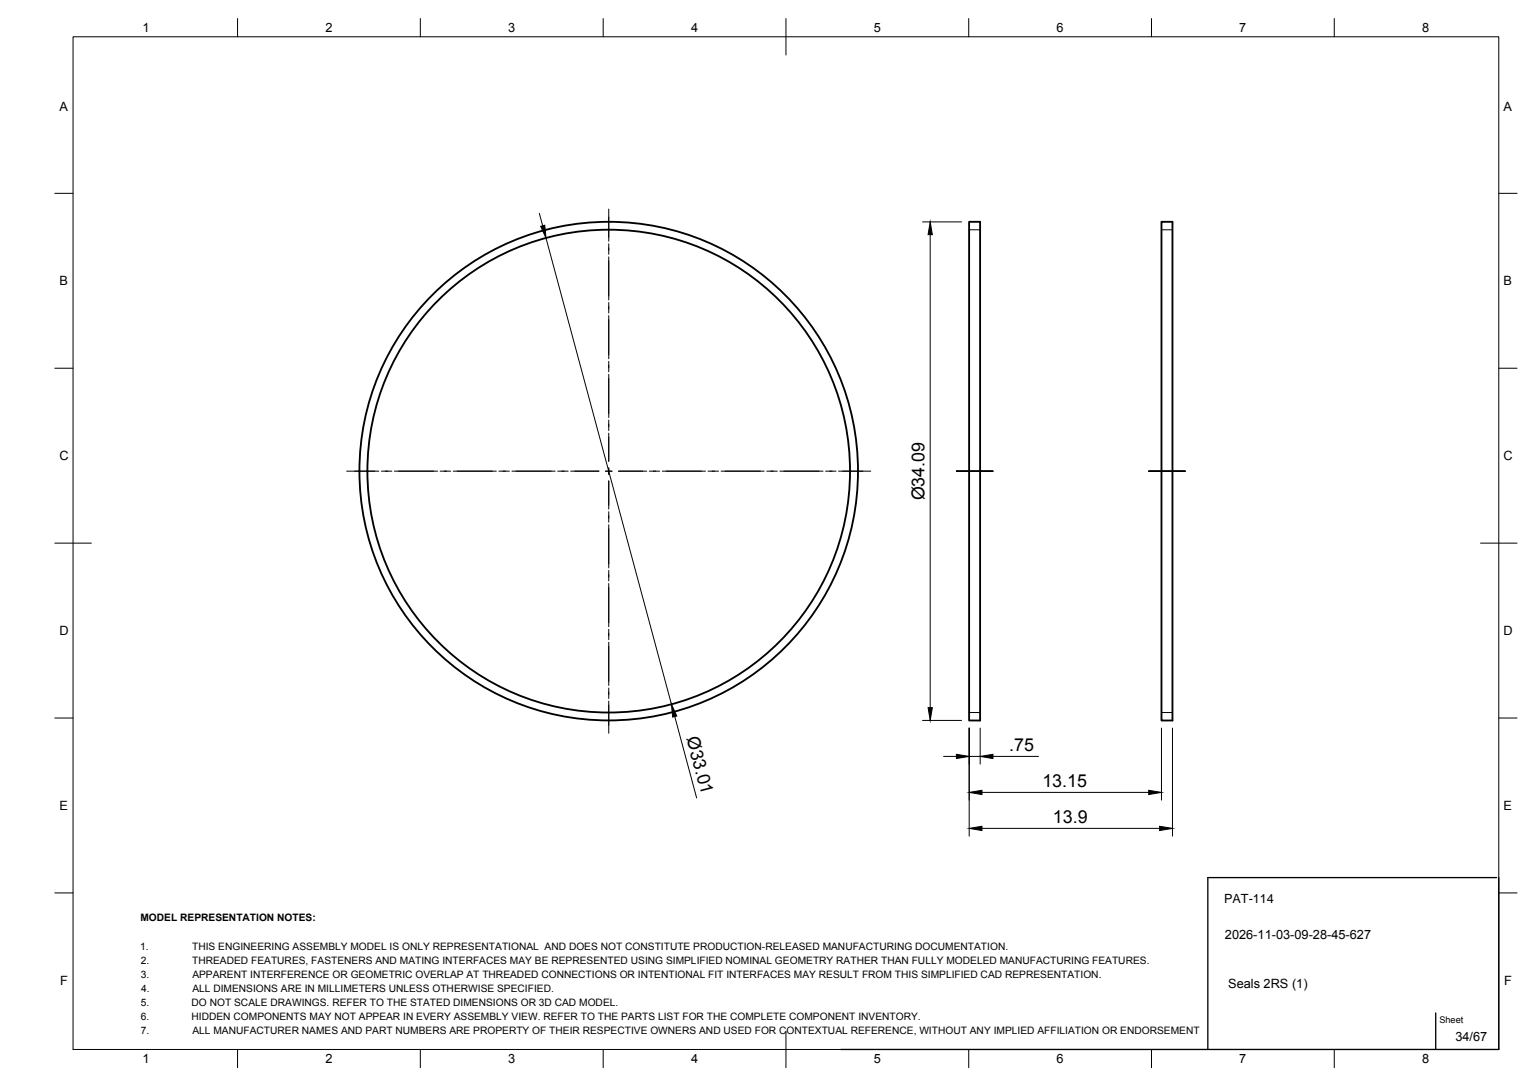
ISO-10303-21;
HEADER;
/* Generated by software containing ST-Developer
 * from STEP Tools, Inc. (www.steptools.com) 
 */

FILE_DESCRIPTION(
/* description */ ('Two-stage gear reducer in split housing'),
/* implementation_level */ '2;1');

FILE_NAME(
/* name */ 'Seals 2RS (1).step',
/* time_stamp */ '2026-10-28T03:22:31-07:00',
/* author */ (''),
/* organization */ (''),
/* preprocessor_version */ 'ST-DEVELOPER v20.2',
/* originating_system */ 'Autodesk Translation Framework v15.17.0.0',
/* authorisation */ '');

FILE_SCHEMA (('AUTOMOTIVE_DESIGN { 1 0 10303 214 3 1 1 }'));
ENDSEC;

DATA;
#10=MECHANICAL_DESIGN_GEOMETRIC_PRESENTATION_REPRESENTATION('',(#1274,#1275),#73366);
#1148=SHAPE_REPRESENTATION_RELATIONSHIP('SRR','None',#73637,#1204);
#1204=ADVANCED_BREP_SHAPE_REPRESENTATION('',(#1344,#1345),#73333);
#1274=STYLED_ITEM('',(#73988),#1344);
#1275=STYLED_ITEM('',(#73988),#1345);
#1344=MANIFOLD_SOLID_BREP('Body1',#16163);
#1345=MANIFOLD_SOLID_BREP('Body2',#16164);
#1533=FACE_BOUND('',#3464,.T.);
#1534=FACE_BOUND('',#3467,.T.);
#1535=FACE_BOUND('',#3470,.T.);
#1536=FACE_BOUND('',#3473,.T.);
#1784=PLANE('',#17657);
#1785=PLANE('',#17662);
#1786=PLANE('',#17665);
#1787=PLANE('',#17670);
#2391=FACE_OUTER_BOUND('',#3463,.T.);
#2392=FACE_OUTER_BOUND('',#3465,.T.);
#2393=FACE_OUTER_BOUND('',#3466,.T.);
#2394=FACE_OUTER_BOUND('',#3468,.T.);
#2395=FACE_OUTER_BOUND('',#3469,.T.);
#2396=FACE_OUTER_BOUND('',#3471,.T.);
#2397=FACE_OUTER_BOUND('',#3472,.T.);
#2398=FACE_OUTER_BOUND('',#3474,.T.);
#3463=EDGE_LOOP('',(#12201));
#3464=EDGE_LOOP('',(#12202));
#3465=EDGE_LOOP('',(#12203,#12204,#12205,#12206));
#3466=EDGE_LOOP('',(#12207));
#3467=EDGE_LOOP('',(#12208));
#3468=EDGE_LOOP('',(#12209,#12210,#12211,#12212));
#3469=EDGE_LOOP('',(#12213));
#3470=EDGE_LOOP('',(#12214));
#3471=EDGE_LOOP('',(#12215,#12216,#12217,#12218));
#3472=EDGE_LOOP('',(#12219));
#3473=EDGE_LOOP('',(#12220));
#3474=EDGE_LOOP('',(#12221,#12222,#12223,#12224));
#4451=LINE('',#25267,#5475);
#4452=LINE('',#25272,#5476);
#4453=LINE('',#25281,#5477);
#4454=LINE('',#25286,#5478);
#5475=VECTOR('',#20553,1.70469);
#5476=VECTOR('',#20560,1.65031);
#5477=VECTOR('',#20571,1.70469);
#5478=VECTOR('',#20578,1.65031);
#6524=CIRCLE('',#17658,1.70469);
#6525=CIRCLE('',#17659,1.65031);
#6526=CIRCLE('',#17661,1.70469);
#6527=CIRCLE('',#17663,1.65031);
#6528=CIRCLE('',#17666,1.70469);
#6529=CIRCLE('',#17667,1.65031);
#6530=CIRCLE('',#17669,1.70469);
#6531=CIRCLE('',#17671,1.65031);
#7405=VERTEX_POINT('',#25260);
#7406=VERTEX_POINT('',#25262);
#7407=VERTEX_POINT('',#25265);
#7408=VERTEX_POINT('',#25269);
#7409=VERTEX_POINT('',#25274);
#7410=VERTEX_POINT('',#25276);
#7411=VERTEX_POINT('',#25279);
#7412=VERTEX_POINT('',#25283);
#9154=EDGE_CURVE('',#7405,#7405,#6524,.T.);
#9155=EDGE_CURVE('',#7406,#7406,#6525,.T.);
#9156=EDGE_CURVE('',#7407,#7407,#6526,.T.);
#9157=EDGE_CURVE('',#7407,#7405,#4451,.T.);
#9158=EDGE_CURVE('',#7408,#7408,#6527,.T.);
#9159=EDGE_CURVE('',#7408,#7406,#4452,.T.);
#9160=EDGE_CURVE('',#7409,#7409,#6528,.T.);
#9161=EDGE_CURVE('',#7410,#7410,#6529,.T.);
#9162=EDGE_CURVE('',#7411,#7411,#6530,.T.);
#9163=EDGE_CURVE('',#7411,#7409,#4453,.T.);
#9164=EDGE_CURVE('',#7412,#7412,#6531,.T.);
#9165=EDGE_CURVE('',#7412,#7410,#4454,.T.);
#12201=ORIENTED_EDGE('',*,*,#9154,.F.);
#12202=ORIENTED_EDGE('',*,*,#9155,.T.);
#12203=ORIENTED_EDGE('',*,*,#9156,.F.);
#12204=ORIENTED_EDGE('',*,*,#9157,.T.);
#12205=ORIENTED_EDGE('',*,*,#9154,.T.);
#12206=ORIENTED_EDGE('',*,*,#9157,.F.);
#12207=ORIENTED_EDGE('',*,*,#9156,.T.);
#12208=ORIENTED_EDGE('',*,*,#9158,.F.);
#12209=ORIENTED_EDGE('',*,*,#9158,.T.);
#12210=ORIENTED_EDGE('',*,*,#9159,.T.);
#12211=ORIENTED_EDGE('',*,*,#9155,.F.);
#12212=ORIENTED_EDGE('',*,*,#9159,.F.);
#12213=ORIENTED_EDGE('',*,*,#9160,.F.);
#12214=ORIENTED_EDGE('',*,*,#9161,.T.);
#12215=ORIENTED_EDGE('',*,*,#9162,.F.);
#12216=ORIENTED_EDGE('',*,*,#9163,.T.);
#12217=ORIENTED_EDGE('',*,*,#9160,.T.);
#12218=ORIENTED_EDGE('',*,*,#9163,.F.);
#12219=ORIENTED_EDGE('',*,*,#9162,.T.);
#12220=ORIENTED_EDGE('',*,*,#9164,.F.);
#12221=ORIENTED_EDGE('',*,*,#9164,.T.);
#12222=ORIENTED_EDGE('',*,*,#9165,.T.);
#12223=ORIENTED_EDGE('',*,*,#9161,.F.);
#12224=ORIENTED_EDGE('',*,*,#9165,.F.);
#15069=CYLINDRICAL_SURFACE('',#17660,1.70469);
#15070=CYLINDRICAL_SURFACE('',#17664,1.65031);
#15071=CYLINDRICAL_SURFACE('',#17668,1.70469);
#15072=CYLINDRICAL_SURFACE('',#17672,1.65031);
#15598=ADVANCED_FACE('',(#2391,#1533),#1784,.T.);
#15599=ADVANCED_FACE('',(#2392),#15069,.T.);
#15600=ADVANCED_FACE('',(#2393,#1534),#1785,.T.);
#15601=ADVANCED_FACE('',(#2394),#15070,.F.);
#15602=ADVANCED_FACE('',(#2395,#1535),#1786,.T.);
#15603=ADVANCED_FACE('',(#2396),#15071,.T.);
#15604=ADVANCED_FACE('',(#2397,#1536),#1787,.T.);
#15605=ADVANCED_FACE('',(#2398),#15072,.F.);
#16163=CLOSED_SHELL('',(#15598,#15599,#15600,#15601));
#16164=CLOSED_SHELL('',(#15602,#15603,#15604,#15605));
#17656=AXIS2_PLACEMENT_3D('',#25258,#20541,#20542);
#17657=AXIS2_PLACEMENT_3D('',#25259,#20543,#20544);
#17658=AXIS2_PLACEMENT_3D('',#25261,#20545,#20546);
#17659=AXIS2_PLACEMENT_3D('',#25263,#20547,#20548);
#17660=AXIS2_PLACEMENT_3D('',#25264,#20549,#20550);
#17661=AXIS2_PLACEMENT_3D('',#25266,#20551,#20552);
#17662=AXIS2_PLACEMENT_3D('',#25268,#20554,#20555);
#17663=AXIS2_PLACEMENT_3D('',#25270,#20556,#20557);
#17664=AXIS2_PLACEMENT_3D('',#25271,#20558,#20559);
#17665=AXIS2_PLACEMENT_3D('',#25273,#20561,#20562);
#17666=AXIS2_PLACEMENT_3D('',#25275,#20563,#20564);
#17667=AXIS2_PLACEMENT_3D('',#25277,#20565,#20566);
#17668=AXIS2_PLACEMENT_3D('',#25278,#20567,#20568);
#17669=AXIS2_PLACEMENT_3D('',#25280,#20569,#20570);
#17670=AXIS2_PLACEMENT_3D('',#25282,#20572,#20573);
#17671=AXIS2_PLACEMENT_3D('',#25284,#20574,#20575);
#17672=AXIS2_PLACEMENT_3D('',#25285,#20576,#20577);
#20541=DIRECTION('axis',(0.,0.,1.));
#20542=DIRECTION('refdir',(1.,0.,0.));
#20543=DIRECTION('center_axis',(0.,1.,0.));
#20544=DIRECTION('ref_axis',(0.,0.,1.));
#20545=DIRECTION('center_axis',(0.,-1.,0.));
#20546=DIRECTION('ref_axis',(1.,0.,0.));
#20547=DIRECTION('center_axis',(0.,-1.,0.));
#20548=DIRECTION('ref_axis',(1.,0.,0.));
#20549=DIRECTION('center_axis',(0.,-1.,0.));
#20550=DIRECTION('ref_axis',(1.,0.,0.));
#20551=DIRECTION('center_axis',(0.,-1.,0.));
#20552=DIRECTION('ref_axis',(1.,0.,0.));
#20553=DIRECTION('',(0.,1.,0.));
#20554=DIRECTION('center_axis',(0.,-1.,0.));
#20555=DIRECTION('ref_axis',(0.,0.,-1.));
#20556=DIRECTION('center_axis',(0.,-1.,0.));
#20557=DIRECTION('ref_axis',(1.,0.,0.));
#20558=DIRECTION('center_axis',(0.,-1.,0.));
#20559=DIRECTION('ref_axis',(1.,0.,0.));
#20560=DIRECTION('',(0.,1.,0.));
#20561=DIRECTION('center_axis',(0.,1.,0.));
#20562=DIRECTION('ref_axis',(0.,0.,1.));
#20563=DIRECTION('center_axis',(0.,-1.,0.));
#20564=DIRECTION('ref_axis',(1.,0.,0.));
#20565=DIRECTION('center_axis',(0.,-1.,0.));
#20566=DIRECTION('ref_axis',(1.,0.,0.));
#20567=DIRECTION('center_axis',(0.,-1.,0.));
#20568=DIRECTION('ref_axis',(1.,0.,0.));
#20569=DIRECTION('center_axis',(0.,-1.,0.));
#20570=DIRECTION('ref_axis',(1.,0.,0.));
#20571=DIRECTION('',(0.,1.,0.));
#20572=DIRECTION('center_axis',(0.,-1.,0.));
#20573=DIRECTION('ref_axis',(0.,0.,-1.));
#20574=DIRECTION('center_axis',(0.,-1.,0.));
#20575=DIRECTION('ref_axis',(1.,0.,0.));
#20576=DIRECTION('center_axis',(0.,-1.,0.));
#20577=DIRECTION('ref_axis',(1.,0.,0.));
#20578=DIRECTION('',(0.,1.,0.));
#25258=CARTESIAN_POINT('',(0.,0.,0.));
#25259=CARTESIAN_POINT('Origin',(1.70469,0.695,0.));
#25260=CARTESIAN_POINT('',(-1.70469,0.695,-2.0876431520385E-16));
#25261=CARTESIAN_POINT('Origin',(0.,0.695,0.));
#25262=CARTESIAN_POINT('',(-1.65031,0.695,-2.02104685910087E-16));
#25263=CARTESIAN_POINT('Origin',(0.,0.695,0.));
#25264=CARTESIAN_POINT('Origin',(0.,0.6575,0.));
#25265=CARTESIAN_POINT('',(-1.70469,0.62,-2.0876431520385E-16));
#25266=CARTESIAN_POINT('Origin',(0.,0.62,0.));
#25267=CARTESIAN_POINT('',(-1.70469,0.6575,-2.0876431520385E-16));
#25268=CARTESIAN_POINT('Origin',(1.65031,0.62,0.));
#25269=CARTESIAN_POINT('',(-1.65031,0.62,-2.02104685910087E-16));
#25270=CARTESIAN_POINT('Origin',(0.,0.62,0.));
#25271=CARTESIAN_POINT('Origin',(0.,0.6575,0.));
#25272=CARTESIAN_POINT('',(-1.65031,0.6575,-2.02104685910087E-16));
#25273=CARTESIAN_POINT('Origin',(1.70469,-0.62,0.));
#25274=CARTESIAN_POINT('',(-1.70469,-0.62,-2.0876431520385E-16));
#25275=CARTESIAN_POINT('Origin',(0.,-0.62,0.));
#25276=CARTESIAN_POINT('',(-1.65031,-0.62,-2.02104685910087E-16));
#25277=CARTESIAN_POINT('Origin',(0.,-0.62,0.));
#25278=CARTESIAN_POINT('Origin',(0.,-0.6575,0.));
#25279=CARTESIAN_POINT('',(-1.70469,-0.695,-2.0876431520385E-16));
#25280=CARTESIAN_POINT('Origin',(0.,-0.695,0.));
#25281=CARTESIAN_POINT('',(-1.70469,-0.6575,-2.0876431520385E-16));
#25282=CARTESIAN_POINT('Origin',(1.65031,-0.695,0.));
#25283=CARTESIAN_POINT('',(-1.65031,-0.695,-2.02104685910087E-16));
#25284=CARTESIAN_POINT('Origin',(0.,-0.695,0.));
#25285=CARTESIAN_POINT('Origin',(0.,-0.6575,0.));
#25286=CARTESIAN_POINT('',(-1.65031,-0.6575,-2.02104685910087E-16));
#73269=UNCERTAINTY_MEASURE_WITH_UNIT(LENGTH_MEASURE(0.001),#73367,
'DISTANCE_ACCURACY_VALUE',
'Maximum model space distance between geometric entities at asserted c
onnectivities');
#73302=UNCERTAINTY_MEASURE_WITH_UNIT(LENGTH_MEASURE(0.001),#73367,
'DISTANCE_ACCURACY_VALUE',
'Maximum model space distance between geometric entities at asserted c
onnectivities');
#73333=(
GEOMETRIC_REPRESENTATION_CONTEXT(3)
GLOBAL_UNCERTAINTY_ASSIGNED_CONTEXT((#73269))
GLOBAL_UNIT_ASSIGNED_CONTEXT((#73367,#73369,#73370))
REPRESENTATION_CONTEXT('','3D')
);
#73366=(
GEOMETRIC_REPRESENTATION_CONTEXT(3)
GLOBAL_UNCERTAINTY_ASSIGNED_CONTEXT((#73302))
GLOBAL_UNIT_ASSIGNED_CONTEXT((#73367,#73369,#73370))
REPRESENTATION_CONTEXT('','3D')
);
#73367=(
LENGTH_UNIT()
NAMED_UNIT(*)
SI_UNIT(.CENTI.,.METRE.)
);
#73369=(
NAMED_UNIT(*)
PLANE_ANGLE_UNIT()
SI_UNIT($,.RADIAN.)
);
#73370=(
NAMED_UNIT(*)
SI_UNIT($,.STERADIAN.)
SOLID_ANGLE_UNIT()
);
#73401=SHAPE_DEFINITION_REPRESENTATION(#73469,#73637);
#73469=PRODUCT_DEFINITION_SHAPE('',$,#73701);
#73637=SHAPE_REPRESENTATION('',(#17656),#73333);
#73670=PRODUCT_DEFINITION_CONTEXT('part definition',#73861,'design');
#73701=PRODUCT_DEFINITION('Seals 2RS (1)','Seals 2RS (1)',#73764,#73670);
#73764=PRODUCT_DEFINITION_FORMATION('',$,#73893);
#73861=APPLICATION_CONTEXT(
'Core Data for Automotive Mechanical Design Process');
#73862=PRODUCT_CONTEXT('part definition',#73861,'mechanical');
#73893=PRODUCT('Seals 2RS (1)','Seals 2RS (1)','Seals 2RS (1)',(#73862));
#73982=COLOUR_RGB('Grey',0.48,0.52,0.57);
#73983=FILL_AREA_STYLE_COLOUR('',#73982);
#73984=FILL_AREA_STYLE('',(#73983));
#73985=SURFACE_STYLE_FILL_AREA(#73984);
#73986=SURFACE_SIDE_STYLE('',(#73985));
#73987=SURFACE_STYLE_USAGE(.BOTH.,#73986);
#73988=PRESENTATION_STYLE_ASSIGNMENT((#73987));
ENDSEC;
END-ISO-10303-21;
